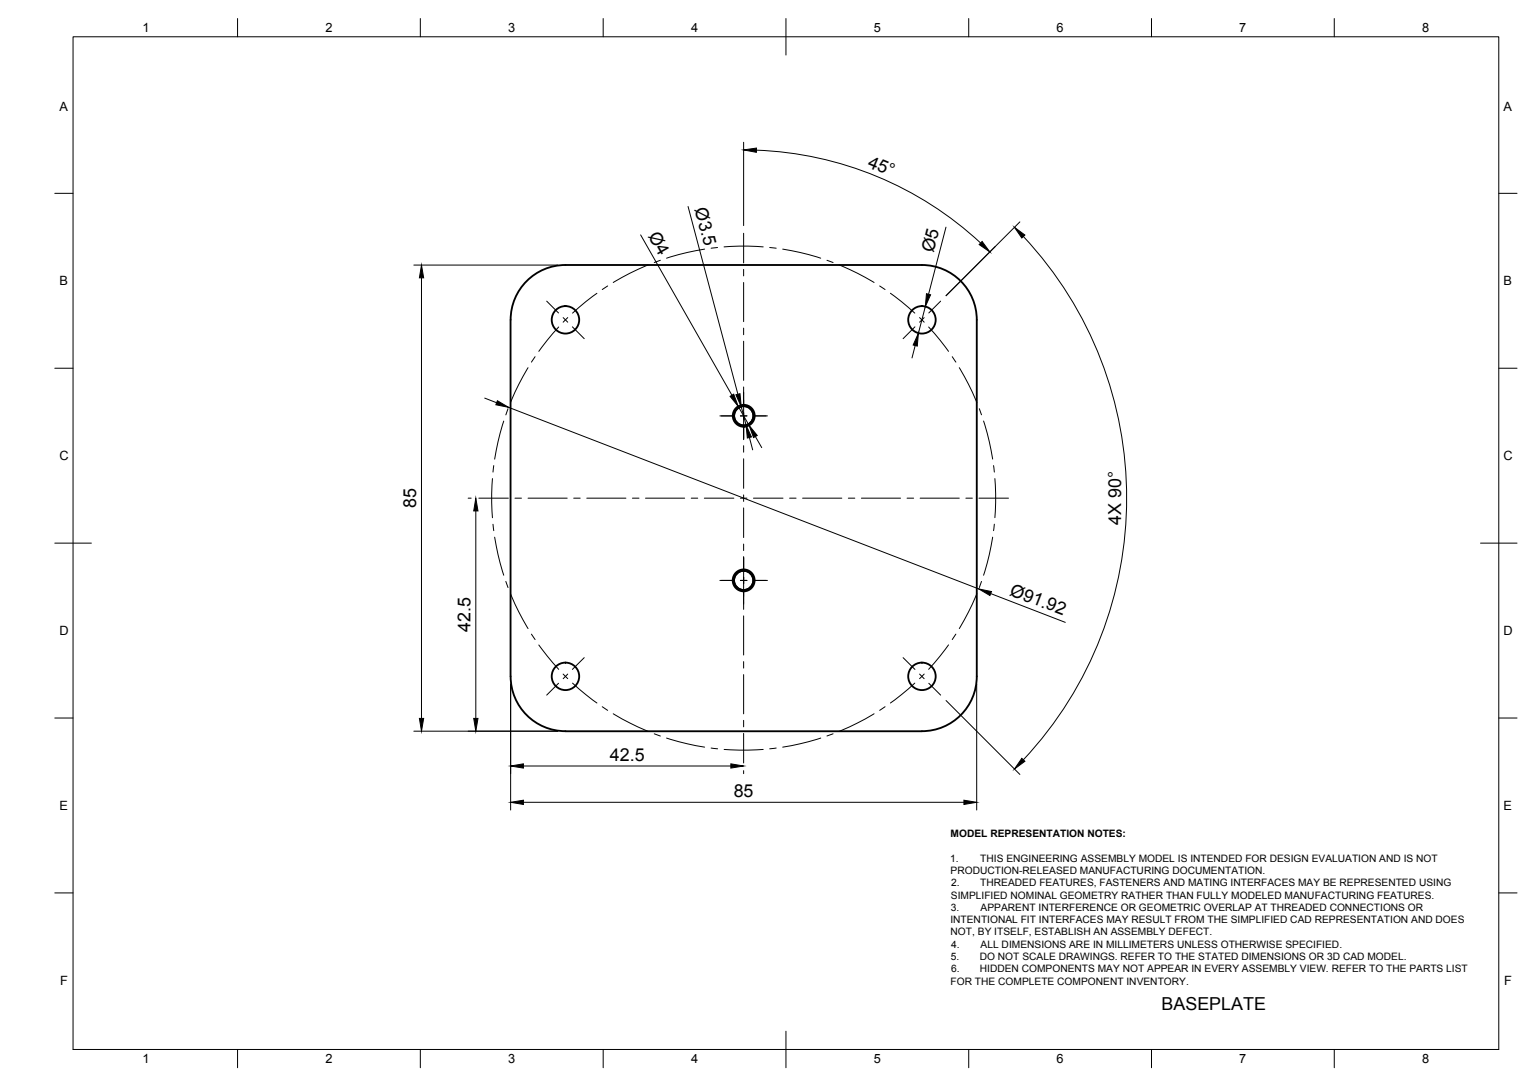
ISO-10303-21;
HEADER;
/* Generated by software containing ST-Developer
 * from STEP Tools, Inc. (www.steptools.com) 
 */

FILE_DESCRIPTION(
/* description */ (''),
/* implementation_level */ '2;1');

FILE_NAME(
/* name */ 'BASEPLATE.step',
/* time_stamp */ '2026-10-06T01:16:10-07:00',
/* author */ (''),
/* organization */ (''),
/* preprocessor_version */ 'ST-DEVELOPER v20.2',
/* originating_system */ 'Autodesk Translation Framework v15.15.0.0',
/* authorisation */ '');

FILE_SCHEMA (('AUTOMOTIVE_DESIGN { 1 0 10303 214 3 1 1 }'));
ENDSEC;

DATA;
#10=MECHANICAL_DESIGN_GEOMETRIC_PRESENTATION_REPRESENTATION('',(#297,#298,#299),#17113);
#221=OPEN_SHELL('',(#5698,#5699));
#222=OPEN_SHELL('',(#5700,#5701));
#239=SHELL_BASED_SURFACE_MODEL('Body2',(#221));
#240=SHELL_BASED_SURFACE_MODEL('Body3',(#222));
#257=CONICAL_SURFACE('',#6271,8.999999999749,0.785398163397448);
#258=CONICAL_SURFACE('',#6274,8.999999999749,0.785398163397448);
#259=CONICAL_SURFACE('',#6277,8.999999999749,0.785398163397448);
#260=CONICAL_SURFACE('',#6280,8.999999999749,0.785398163397448);
#265=SHAPE_REPRESENTATION_RELATIONSHIP('SRR','None',#17187,#281);
#281=ADVANCED_BREP_SHAPE_REPRESENTATION('',(#331),#17094);
#297=STYLED_ITEM('',(#17298),#331);
#298=STYLED_ITEM('',(#17298),#239);
#299=STYLED_ITEM('',(#17298),#240);
#331=MANIFOLD_SOLID_BREP('Body1',#6017);
#352=CYLINDRICAL_SURFACE('',#6254,2.5);
#353=CYLINDRICAL_SURFACE('',#6266,2.5);
#354=CYLINDRICAL_SURFACE('',#6267,2.5);
#355=CYLINDRICAL_SURFACE('',#6268,2.5);
#356=CYLINDRICAL_SURFACE('',#6269,1.75);
#357=CYLINDRICAL_SURFACE('',#6270,1.75);
#358=CYLINDRICAL_SURFACE('',#6284,10.);
#359=CYLINDRICAL_SURFACE('',#6286,10.);
#360=CYLINDRICAL_SURFACE('',#6288,10.);
#361=CYLINDRICAL_SURFACE('',#6290,10.);
#362=CYLINDRICAL_SURFACE('',#6291,2.);
#363=CYLINDRICAL_SURFACE('',#6296,2.);
#514=FACE_BOUND('',#1397,.T.);
#515=FACE_BOUND('',#1398,.T.);
#516=FACE_BOUND('',#1399,.T.);
#517=FACE_BOUND('',#1400,.T.);
#518=FACE_BOUND('',#1401,.T.);
#519=FACE_BOUND('',#1402,.T.);
#520=FACE_BOUND('',#1405,.T.);
#521=FACE_BOUND('',#1406,.T.);
#522=FACE_BOUND('',#1407,.T.);
#523=FACE_BOUND('',#1408,.T.);
#524=FACE_BOUND('',#1409,.T.);
#525=FACE_BOUND('',#1410,.T.);
#526=FACE_BOUND('',#1434,.T.);
#527=FACE_BOUND('',#1437,.T.);
#648=CIRCLE('',#6244,10.);
#649=CIRCLE('',#6245,10.);
#650=CIRCLE('',#6246,10.);
#651=CIRCLE('',#6247,10.);
#652=CIRCLE('',#6248,2.5);
#653=CIRCLE('',#6249,2.5);
#654=CIRCLE('',#6250,2.5);
#655=CIRCLE('',#6251,1.75);
#656=CIRCLE('',#6252,1.75);
#657=CIRCLE('',#6253,2.5);
#658=CIRCLE('',#6255,2.5);
#659=CIRCLE('',#6257,8.);
#660=CIRCLE('',#6258,8.);
#661=CIRCLE('',#6259,8.);
#662=CIRCLE('',#6260,8.);
#663=CIRCLE('',#6261,2.5);
#664=CIRCLE('',#6262,2.5);
#665=CIRCLE('',#6263,2.5);
#666=CIRCLE('',#6264,1.75);
#667=CIRCLE('',#6265,1.75);
#668=CIRCLE('',#6272,10.);
#669=CIRCLE('',#6275,10.);
#670=CIRCLE('',#6278,10.);
#671=CIRCLE('',#6281,10.);
#672=CIRCLE('',#6292,2.);
#673=CIRCLE('',#6293,2.);
#674=CIRCLE('',#6295,1.75);
#675=CIRCLE('',#6297,2.);
#676=CIRCLE('',#6298,2.);
#677=CIRCLE('',#6300,1.75);
#1026=FACE_OUTER_BOUND('',#1396,.T.);
#1027=FACE_OUTER_BOUND('',#1403,.T.);
#1028=FACE_OUTER_BOUND('',#1404,.T.);
#1029=FACE_OUTER_BOUND('',#1411,.T.);
#1030=FACE_OUTER_BOUND('',#1412,.T.);
#1031=FACE_OUTER_BOUND('',#1413,.T.);
#1032=FACE_OUTER_BOUND('',#1414,.T.);
#1033=FACE_OUTER_BOUND('',#1415,.T.);
#1034=FACE_OUTER_BOUND('',#1416,.T.);
#1035=FACE_OUTER_BOUND('',#1417,.T.);
#1036=FACE_OUTER_BOUND('',#1418,.T.);
#1037=FACE_OUTER_BOUND('',#1419,.T.);
#1038=FACE_OUTER_BOUND('',#1420,.T.);
#1039=FACE_OUTER_BOUND('',#1421,.T.);
#1040=FACE_OUTER_BOUND('',#1422,.T.);
#1041=FACE_OUTER_BOUND('',#1423,.T.);
#1042=FACE_OUTER_BOUND('',#1424,.T.);
#1043=FACE_OUTER_BOUND('',#1425,.T.);
#1044=FACE_OUTER_BOUND('',#1426,.T.);
#1045=FACE_OUTER_BOUND('',#1427,.T.);
#1046=FACE_OUTER_BOUND('',#1428,.T.);
#1047=FACE_OUTER_BOUND('',#1429,.T.);
#1048=FACE_OUTER_BOUND('',#1430,.T.);
#1049=FACE_OUTER_BOUND('',#1431,.T.);
#1050=FACE_OUTER_BOUND('',#1432,.T.);
#1051=FACE_OUTER_BOUND('',#1433,.T.);
#1052=FACE_OUTER_BOUND('',#1435,.T.);
#1053=FACE_OUTER_BOUND('',#1436,.T.);
#1396=EDGE_LOOP('',(#3996,#3997,#3998,#3999,#4000,#4001,#4002,#4003));
#1397=EDGE_LOOP('',(#4004));
#1398=EDGE_LOOP('',(#4005));
#1399=EDGE_LOOP('',(#4006));
#1400=EDGE_LOOP('',(#4007));
#1401=EDGE_LOOP('',(#4008));
#1402=EDGE_LOOP('',(#4009));
#1403=EDGE_LOOP('',(#4010,#4011,#4012,#4013));
#1404=EDGE_LOOP('',(#4014,#4015,#4016,#4017,#4018,#4019,#4020,#4021));
#1405=EDGE_LOOP('',(#4022));
#1406=EDGE_LOOP('',(#4023));
#1407=EDGE_LOOP('',(#4024));
#1408=EDGE_LOOP('',(#4025));
#1409=EDGE_LOOP('',(#4026));
#1410=EDGE_LOOP('',(#4027));
#1411=EDGE_LOOP('',(#4028,#4029,#4030,#4031));
#1412=EDGE_LOOP('',(#4032,#4033,#4034,#4035));
#1413=EDGE_LOOP('',(#4036,#4037,#4038,#4039));
#1414=EDGE_LOOP('',(#4040,#4041,#4042,#4043));
#1415=EDGE_LOOP('',(#4044,#4045,#4046,#4047));
#1416=EDGE_LOOP('',(#4048,#4049,#4050,#4051));
#1417=EDGE_LOOP('',(#4052,#4053,#4054,#4055));
#1418=EDGE_LOOP('',(#4056,#4057,#4058,#4059));
#1419=EDGE_LOOP('',(#4060,#4061,#4062,#4063));
#1420=EDGE_LOOP('',(#4064,#4065,#4066,#4067));
#1421=EDGE_LOOP('',(#4068,#4069,#4070,#4071));
#1422=EDGE_LOOP('',(#4072,#4073,#4074,#4075));
#1423=EDGE_LOOP('',(#4076,#4077,#4078,#4079));
#1424=EDGE_LOOP('',(#4080,#4081,#4082,#4083));
#1425=EDGE_LOOP('',(#4084,#4085,#4086,#4087));
#1426=EDGE_LOOP('',(#4088,#4089,#4090,#4091));
#1427=EDGE_LOOP('',(#4092,#4093,#4094,#4095));
#1428=EDGE_LOOP('',(#4096,#4097,#4098,#4099));
#1429=EDGE_LOOP('',(#4100,#4101,#4102,#4103));
#1430=EDGE_LOOP('',(#4104,#4105,#4106,#4107));
#1431=EDGE_LOOP('',(#4108,#4109,#4110,#4111));
#1432=EDGE_LOOP('',(#4112,#4113,#4114,#4115));
#1433=EDGE_LOOP('',(#4116));
#1434=EDGE_LOOP('',(#4117));
#1435=EDGE_LOOP('',(#4118,#4119,#4120,#4121));
#1436=EDGE_LOOP('',(#4122));
#1437=EDGE_LOOP('',(#4123));
#1888=LINE('',#8970,#2249);
#1889=LINE('',#8974,#2250);
#1890=LINE('',#8978,#2251);
#1891=LINE('',#8981,#2252);
#1892=LINE('',#8996,#2253);
#1893=LINE('',#9003,#2254);
#1894=LINE('',#9007,#2255);
#1895=LINE('',#9011,#2256);
#1896=LINE('',#9014,#2257);
#1897=LINE('',#9026,#2258);
#1898=LINE('',#9028,#2259);
#1899=LINE('',#9030,#2260);
#1900=LINE('',#9032,#2261);
#1901=LINE('',#9034,#2262);
#1902=LINE('',#9037,#2263);
#1903=LINE('',#9040,#2264);
#1904=LINE('',#9043,#2265);
#1905=LINE('',#9044,#2266);
#1906=LINE('',#9048,#2267);
#1907=LINE('',#9051,#2268);
#1908=LINE('',#9052,#2269);
#1909=LINE('',#9056,#2270);
#1910=LINE('',#9059,#2271);
#1911=LINE('',#9060,#2272);
#1912=LINE('',#9064,#2273);
#1913=LINE('',#9066,#2274);
#1914=LINE('',#9068,#2275);
#1915=LINE('',#9069,#2276);
#1916=LINE('',#9071,#2277);
#1917=LINE('',#9073,#2278);
#1918=LINE('',#9075,#2279);
#1919=LINE('',#9077,#2280);
#1920=LINE('',#9079,#2281);
#1921=LINE('',#9081,#2282);
#1922=LINE('',#9087,#2283);
#1923=LINE('',#9096,#2284);
#2249=VECTOR('',#7078,65.);
#2250=VECTOR('',#7081,65.);
#2251=VECTOR('',#7084,65.);
#2252=VECTOR('',#7087,65.);
#2253=VECTOR('',#7102,2.5);
#2254=VECTOR('',#7109,64.99999997841);
#2255=VECTOR('',#7112,64.99999997841);
#2256=VECTOR('',#7115,64.99999997841);
#2257=VECTOR('',#7118,64.99999997841);
#2258=VECTOR('',#7131,2.5);
#2259=VECTOR('',#7134,2.5);
#2260=VECTOR('',#7137,2.5);
#2261=VECTOR('',#7140,1.75);
#2262=VECTOR('',#7143,1.75);
#2263=VECTOR('',#7146,2.82842712475481);
#2264=VECTOR('',#7149,2.82842712476101);
#2265=VECTOR('',#7152,64.99999997975);
#2266=VECTOR('',#7153,2.82842712475481);
#2267=VECTOR('',#7158,2.82842712476081);
#2268=VECTOR('',#7161,64.99999997975);
#2269=VECTOR('',#7162,2.82842712475481);
#2270=VECTOR('',#7167,2.82842712476101);
#2271=VECTOR('',#7170,64.99999997975);
#2272=VECTOR('',#7171,2.82842712475481);
#2273=VECTOR('',#7176,2.82842712476081);
#2274=VECTOR('',#7179,64.99999997975);
#2275=VECTOR('',#7182,4.000000000157);
#2276=VECTOR('',#7183,4.00000000009);
#2277=VECTOR('',#7186,4.000000000157);
#2278=VECTOR('',#7189,4.00000000009);
#2279=VECTOR('',#7192,4.000000000157);
#2280=VECTOR('',#7195,4.00000000009);
#2281=VECTOR('',#7198,4.000000000157);
#2282=VECTOR('',#7201,4.00000000009);
#2283=VECTOR('',#7208,2.);
#2284=VECTOR('',#7219,2.);
#2608=VERTEX_POINT('',#8966);
#2609=VERTEX_POINT('',#8967);
#2610=VERTEX_POINT('',#8969);
#2611=VERTEX_POINT('',#8971);
#2612=VERTEX_POINT('',#8973);
#2613=VERTEX_POINT('',#8975);
#2614=VERTEX_POINT('',#8977);
#2615=VERTEX_POINT('',#8979);
#2616=VERTEX_POINT('',#8982);
#2617=VERTEX_POINT('',#8984);
#2618=VERTEX_POINT('',#8986);
#2619=VERTEX_POINT('',#8988);
#2620=VERTEX_POINT('',#8990);
#2621=VERTEX_POINT('',#8992);
#2622=VERTEX_POINT('',#8995);
#2623=VERTEX_POINT('',#8999);
#2624=VERTEX_POINT('',#9000);
#2625=VERTEX_POINT('',#9002);
#2626=VERTEX_POINT('',#9004);
#2627=VERTEX_POINT('',#9006);
#2628=VERTEX_POINT('',#9008);
#2629=VERTEX_POINT('',#9010);
#2630=VERTEX_POINT('',#9012);
#2631=VERTEX_POINT('',#9015);
#2632=VERTEX_POINT('',#9017);
#2633=VERTEX_POINT('',#9019);
#2634=VERTEX_POINT('',#9021);
#2635=VERTEX_POINT('',#9023);
#2636=VERTEX_POINT('',#9036);
#2637=VERTEX_POINT('',#9038);
#2638=VERTEX_POINT('',#9042);
#2639=VERTEX_POINT('',#9046);
#2640=VERTEX_POINT('',#9050);
#2641=VERTEX_POINT('',#9054);
#2642=VERTEX_POINT('',#9058);
#2643=VERTEX_POINT('',#9062);
#2644=VERTEX_POINT('',#9084);
#2645=VERTEX_POINT('',#9086);
#2646=VERTEX_POINT('',#9090);
#2647=VERTEX_POINT('',#9093);
#2648=VERTEX_POINT('',#9095);
#2649=VERTEX_POINT('',#9099);
#3144=EDGE_CURVE('',#2608,#2609,#648,.T.);
#3145=EDGE_CURVE('',#2610,#2608,#1888,.T.);
#3146=EDGE_CURVE('',#2611,#2610,#649,.T.);
#3147=EDGE_CURVE('',#2612,#2611,#1889,.T.);
#3148=EDGE_CURVE('',#2613,#2612,#650,.T.);
#3149=EDGE_CURVE('',#2614,#2613,#1890,.T.);
#3150=EDGE_CURVE('',#2615,#2614,#651,.T.);
#3151=EDGE_CURVE('',#2609,#2615,#1891,.T.);
#3152=EDGE_CURVE('',#2616,#2616,#652,.T.);
#3153=EDGE_CURVE('',#2617,#2617,#653,.T.);
#3154=EDGE_CURVE('',#2618,#2618,#654,.T.);
#3155=EDGE_CURVE('',#2619,#2619,#655,.T.);
#3156=EDGE_CURVE('',#2620,#2620,#656,.T.);
#3157=EDGE_CURVE('',#2621,#2621,#657,.T.);
#3158=EDGE_CURVE('',#2621,#2622,#1892,.T.);
#3159=EDGE_CURVE('',#2622,#2622,#658,.T.);
#3160=EDGE_CURVE('',#2623,#2624,#659,.T.);
#3161=EDGE_CURVE('',#2624,#2625,#1893,.T.);
#3162=EDGE_CURVE('',#2625,#2626,#660,.T.);
#3163=EDGE_CURVE('',#2626,#2627,#1894,.T.);
#3164=EDGE_CURVE('',#2627,#2628,#661,.T.);
#3165=EDGE_CURVE('',#2628,#2629,#1895,.T.);
#3166=EDGE_CURVE('',#2629,#2630,#662,.T.);
#3167=EDGE_CURVE('',#2630,#2623,#1896,.T.);
#3168=EDGE_CURVE('',#2631,#2631,#663,.T.);
#3169=EDGE_CURVE('',#2632,#2632,#664,.T.);
#3170=EDGE_CURVE('',#2633,#2633,#665,.T.);
#3171=EDGE_CURVE('',#2634,#2634,#666,.T.);
#3172=EDGE_CURVE('',#2635,#2635,#667,.T.);
#3173=EDGE_CURVE('',#2616,#2631,#1897,.T.);
#3174=EDGE_CURVE('',#2617,#2632,#1898,.T.);
#3175=EDGE_CURVE('',#2618,#2633,#1899,.T.);
#3176=EDGE_CURVE('',#2619,#2634,#1900,.T.);
#3177=EDGE_CURVE('',#2620,#2635,#1901,.T.);
#3178=EDGE_CURVE('',#2623,#2636,#1902,.T.);
#3179=EDGE_CURVE('',#2636,#2637,#668,.T.);
#3180=EDGE_CURVE('',#2624,#2637,#1903,.T.);
#3181=EDGE_CURVE('',#2637,#2638,#1904,.T.);
#3182=EDGE_CURVE('',#2625,#2638,#1905,.T.);
#3183=EDGE_CURVE('',#2638,#2639,#669,.T.);
#3184=EDGE_CURVE('',#2626,#2639,#1906,.T.);
#3185=EDGE_CURVE('',#2639,#2640,#1907,.T.);
#3186=EDGE_CURVE('',#2627,#2640,#1908,.T.);
#3187=EDGE_CURVE('',#2640,#2641,#670,.T.);
#3188=EDGE_CURVE('',#2628,#2641,#1909,.T.);
#3189=EDGE_CURVE('',#2641,#2642,#1910,.T.);
#3190=EDGE_CURVE('',#2629,#2642,#1911,.T.);
#3191=EDGE_CURVE('',#2642,#2643,#671,.T.);
#3192=EDGE_CURVE('',#2630,#2643,#1912,.T.);
#3193=EDGE_CURVE('',#2643,#2636,#1913,.T.);
#3194=EDGE_CURVE('',#2612,#2643,#1914,.T.);
#3195=EDGE_CURVE('',#2611,#2636,#1915,.T.);
#3196=EDGE_CURVE('',#2610,#2637,#1916,.T.);
#3197=EDGE_CURVE('',#2608,#2638,#1917,.T.);
#3198=EDGE_CURVE('',#2609,#2639,#1918,.T.);
#3199=EDGE_CURVE('',#2615,#2640,#1919,.T.);
#3200=EDGE_CURVE('',#2614,#2641,#1920,.T.);
#3201=EDGE_CURVE('',#2613,#2642,#1921,.T.);
#3202=EDGE_CURVE('',#2644,#2644,#672,.T.);
#3203=EDGE_CURVE('',#2644,#2645,#1922,.T.);
#3204=EDGE_CURVE('',#2645,#2645,#673,.T.);
#3205=EDGE_CURVE('',#2646,#2646,#674,.T.);
#3206=EDGE_CURVE('',#2647,#2647,#675,.T.);
#3207=EDGE_CURVE('',#2647,#2648,#1923,.T.);
#3208=EDGE_CURVE('',#2648,#2648,#676,.T.);
#3209=EDGE_CURVE('',#2649,#2649,#677,.T.);
#3996=ORIENTED_EDGE('',*,*,#3144,.F.);
#3997=ORIENTED_EDGE('',*,*,#3145,.F.);
#3998=ORIENTED_EDGE('',*,*,#3146,.F.);
#3999=ORIENTED_EDGE('',*,*,#3147,.F.);
#4000=ORIENTED_EDGE('',*,*,#3148,.F.);
#4001=ORIENTED_EDGE('',*,*,#3149,.F.);
#4002=ORIENTED_EDGE('',*,*,#3150,.F.);
#4003=ORIENTED_EDGE('',*,*,#3151,.F.);
#4004=ORIENTED_EDGE('',*,*,#3152,.F.);
#4005=ORIENTED_EDGE('',*,*,#3153,.F.);
#4006=ORIENTED_EDGE('',*,*,#3154,.F.);
#4007=ORIENTED_EDGE('',*,*,#3155,.F.);
#4008=ORIENTED_EDGE('',*,*,#3156,.F.);
#4009=ORIENTED_EDGE('',*,*,#3157,.F.);
#4010=ORIENTED_EDGE('',*,*,#3157,.T.);
#4011=ORIENTED_EDGE('',*,*,#3158,.T.);
#4012=ORIENTED_EDGE('',*,*,#3159,.F.);
#4013=ORIENTED_EDGE('',*,*,#3158,.F.);
#4014=ORIENTED_EDGE('',*,*,#3160,.T.);
#4015=ORIENTED_EDGE('',*,*,#3161,.T.);
#4016=ORIENTED_EDGE('',*,*,#3162,.T.);
#4017=ORIENTED_EDGE('',*,*,#3163,.T.);
#4018=ORIENTED_EDGE('',*,*,#3164,.T.);
#4019=ORIENTED_EDGE('',*,*,#3165,.T.);
#4020=ORIENTED_EDGE('',*,*,#3166,.T.);
#4021=ORIENTED_EDGE('',*,*,#3167,.T.);
#4022=ORIENTED_EDGE('',*,*,#3168,.T.);
#4023=ORIENTED_EDGE('',*,*,#3169,.T.);
#4024=ORIENTED_EDGE('',*,*,#3170,.T.);
#4025=ORIENTED_EDGE('',*,*,#3171,.T.);
#4026=ORIENTED_EDGE('',*,*,#3172,.T.);
#4027=ORIENTED_EDGE('',*,*,#3159,.T.);
#4028=ORIENTED_EDGE('',*,*,#3152,.T.);
#4029=ORIENTED_EDGE('',*,*,#3173,.T.);
#4030=ORIENTED_EDGE('',*,*,#3168,.F.);
#4031=ORIENTED_EDGE('',*,*,#3173,.F.);
#4032=ORIENTED_EDGE('',*,*,#3153,.T.);
#4033=ORIENTED_EDGE('',*,*,#3174,.T.);
#4034=ORIENTED_EDGE('',*,*,#3169,.F.);
#4035=ORIENTED_EDGE('',*,*,#3174,.F.);
#4036=ORIENTED_EDGE('',*,*,#3154,.T.);
#4037=ORIENTED_EDGE('',*,*,#3175,.T.);
#4038=ORIENTED_EDGE('',*,*,#3170,.F.);
#4039=ORIENTED_EDGE('',*,*,#3175,.F.);
#4040=ORIENTED_EDGE('',*,*,#3155,.T.);
#4041=ORIENTED_EDGE('',*,*,#3176,.T.);
#4042=ORIENTED_EDGE('',*,*,#3171,.F.);
#4043=ORIENTED_EDGE('',*,*,#3176,.F.);
#4044=ORIENTED_EDGE('',*,*,#3156,.T.);
#4045=ORIENTED_EDGE('',*,*,#3177,.T.);
#4046=ORIENTED_EDGE('',*,*,#3172,.F.);
#4047=ORIENTED_EDGE('',*,*,#3177,.F.);
#4048=ORIENTED_EDGE('',*,*,#3160,.F.);
#4049=ORIENTED_EDGE('',*,*,#3178,.T.);
#4050=ORIENTED_EDGE('',*,*,#3179,.T.);
#4051=ORIENTED_EDGE('',*,*,#3180,.F.);
#4052=ORIENTED_EDGE('',*,*,#3161,.F.);
#4053=ORIENTED_EDGE('',*,*,#3180,.T.);
#4054=ORIENTED_EDGE('',*,*,#3181,.T.);
#4055=ORIENTED_EDGE('',*,*,#3182,.F.);
#4056=ORIENTED_EDGE('',*,*,#3162,.F.);
#4057=ORIENTED_EDGE('',*,*,#3182,.T.);
#4058=ORIENTED_EDGE('',*,*,#3183,.T.);
#4059=ORIENTED_EDGE('',*,*,#3184,.F.);
#4060=ORIENTED_EDGE('',*,*,#3163,.F.);
#4061=ORIENTED_EDGE('',*,*,#3184,.T.);
#4062=ORIENTED_EDGE('',*,*,#3185,.T.);
#4063=ORIENTED_EDGE('',*,*,#3186,.F.);
#4064=ORIENTED_EDGE('',*,*,#3164,.F.);
#4065=ORIENTED_EDGE('',*,*,#3186,.T.);
#4066=ORIENTED_EDGE('',*,*,#3187,.T.);
#4067=ORIENTED_EDGE('',*,*,#3188,.F.);
#4068=ORIENTED_EDGE('',*,*,#3165,.F.);
#4069=ORIENTED_EDGE('',*,*,#3188,.T.);
#4070=ORIENTED_EDGE('',*,*,#3189,.T.);
#4071=ORIENTED_EDGE('',*,*,#3190,.F.);
#4072=ORIENTED_EDGE('',*,*,#3166,.F.);
#4073=ORIENTED_EDGE('',*,*,#3190,.T.);
#4074=ORIENTED_EDGE('',*,*,#3191,.T.);
#4075=ORIENTED_EDGE('',*,*,#3192,.F.);
#4076=ORIENTED_EDGE('',*,*,#3167,.F.);
#4077=ORIENTED_EDGE('',*,*,#3192,.T.);
#4078=ORIENTED_EDGE('',*,*,#3193,.T.);
#4079=ORIENTED_EDGE('',*,*,#3178,.F.);
#4080=ORIENTED_EDGE('',*,*,#3193,.F.);
#4081=ORIENTED_EDGE('',*,*,#3194,.F.);
#4082=ORIENTED_EDGE('',*,*,#3147,.T.);
#4083=ORIENTED_EDGE('',*,*,#3195,.T.);
#4084=ORIENTED_EDGE('',*,*,#3179,.F.);
#4085=ORIENTED_EDGE('',*,*,#3195,.F.);
#4086=ORIENTED_EDGE('',*,*,#3146,.T.);
#4087=ORIENTED_EDGE('',*,*,#3196,.T.);
#4088=ORIENTED_EDGE('',*,*,#3181,.F.);
#4089=ORIENTED_EDGE('',*,*,#3196,.F.);
#4090=ORIENTED_EDGE('',*,*,#3145,.T.);
#4091=ORIENTED_EDGE('',*,*,#3197,.T.);
#4092=ORIENTED_EDGE('',*,*,#3183,.F.);
#4093=ORIENTED_EDGE('',*,*,#3197,.F.);
#4094=ORIENTED_EDGE('',*,*,#3144,.T.);
#4095=ORIENTED_EDGE('',*,*,#3198,.T.);
#4096=ORIENTED_EDGE('',*,*,#3185,.F.);
#4097=ORIENTED_EDGE('',*,*,#3198,.F.);
#4098=ORIENTED_EDGE('',*,*,#3151,.T.);
#4099=ORIENTED_EDGE('',*,*,#3199,.T.);
#4100=ORIENTED_EDGE('',*,*,#3187,.F.);
#4101=ORIENTED_EDGE('',*,*,#3199,.F.);
#4102=ORIENTED_EDGE('',*,*,#3150,.T.);
#4103=ORIENTED_EDGE('',*,*,#3200,.T.);
#4104=ORIENTED_EDGE('',*,*,#3189,.F.);
#4105=ORIENTED_EDGE('',*,*,#3200,.F.);
#4106=ORIENTED_EDGE('',*,*,#3149,.T.);
#4107=ORIENTED_EDGE('',*,*,#3201,.T.);
#4108=ORIENTED_EDGE('',*,*,#3191,.F.);
#4109=ORIENTED_EDGE('',*,*,#3201,.F.);
#4110=ORIENTED_EDGE('',*,*,#3148,.T.);
#4111=ORIENTED_EDGE('',*,*,#3194,.T.);
#4112=ORIENTED_EDGE('',*,*,#3202,.F.);
#4113=ORIENTED_EDGE('',*,*,#3203,.T.);
#4114=ORIENTED_EDGE('',*,*,#3204,.T.);
#4115=ORIENTED_EDGE('',*,*,#3203,.F.);
#4116=ORIENTED_EDGE('',*,*,#3204,.F.);
#4117=ORIENTED_EDGE('',*,*,#3205,.F.);
#4118=ORIENTED_EDGE('',*,*,#3206,.F.);
#4119=ORIENTED_EDGE('',*,*,#3207,.T.);
#4120=ORIENTED_EDGE('',*,*,#3208,.T.);
#4121=ORIENTED_EDGE('',*,*,#3207,.F.);
#4122=ORIENTED_EDGE('',*,*,#3208,.F.);
#4123=ORIENTED_EDGE('',*,*,#3209,.F.);
#5516=PLANE('',#6243);
#5517=PLANE('',#6256);
#5518=PLANE('',#6273);
#5519=PLANE('',#6276);
#5520=PLANE('',#6279);
#5521=PLANE('',#6282);
#5522=PLANE('',#6283);
#5523=PLANE('',#6285);
#5524=PLANE('',#6287);
#5525=PLANE('',#6289);
#5526=PLANE('',#6294);
#5527=PLANE('',#6299);
#5674=ADVANCED_FACE('',(#1026,#514,#515,#516,#517,#518,#519),#5516,.F.);
#5675=ADVANCED_FACE('',(#1027),#352,.F.);
#5676=ADVANCED_FACE('',(#1028,#520,#521,#522,#523,#524,#525),#5517,.T.);
#5677=ADVANCED_FACE('',(#1029),#353,.F.);
#5678=ADVANCED_FACE('',(#1030),#354,.F.);
#5679=ADVANCED_FACE('',(#1031),#355,.F.);
#5680=ADVANCED_FACE('',(#1032),#356,.F.);
#5681=ADVANCED_FACE('',(#1033),#357,.F.);
#5682=ADVANCED_FACE('',(#1034),#257,.T.);
#5683=ADVANCED_FACE('',(#1035),#5518,.T.);
#5684=ADVANCED_FACE('',(#1036),#258,.T.);
#5685=ADVANCED_FACE('',(#1037),#5519,.T.);
#5686=ADVANCED_FACE('',(#1038),#259,.T.);
#5687=ADVANCED_FACE('',(#1039),#5520,.T.);
#5688=ADVANCED_FACE('',(#1040),#260,.T.);
#5689=ADVANCED_FACE('',(#1041),#5521,.T.);
#5690=ADVANCED_FACE('',(#1042),#5522,.T.);
#5691=ADVANCED_FACE('',(#1043),#358,.T.);
#5692=ADVANCED_FACE('',(#1044),#5523,.T.);
#5693=ADVANCED_FACE('',(#1045),#359,.T.);
#5694=ADVANCED_FACE('',(#1046),#5524,.T.);
#5695=ADVANCED_FACE('',(#1047),#360,.T.);
#5696=ADVANCED_FACE('',(#1048),#5525,.T.);
#5697=ADVANCED_FACE('',(#1049),#361,.T.);
#5698=ADVANCED_FACE('',(#1050),#362,.T.);
#5699=ADVANCED_FACE('',(#1051,#526),#5526,.F.);
#5700=ADVANCED_FACE('',(#1052),#363,.T.);
#5701=ADVANCED_FACE('',(#1053,#527),#5527,.F.);
#6017=CLOSED_SHELL('',(#5674,#5675,#5676,#5677,#5678,#5679,#5680,#5681,
#5682,#5683,#5684,#5685,#5686,#5687,#5688,#5689,#5690,#5691,#5692,#5693,
#5694,#5695,#5696,#5697));
#6242=AXIS2_PLACEMENT_3D('',#8964,#7072,#7073);
#6243=AXIS2_PLACEMENT_3D('',#8965,#7074,#7075);
#6244=AXIS2_PLACEMENT_3D('',#8968,#7076,#7077);
#6245=AXIS2_PLACEMENT_3D('',#8972,#7079,#7080);
#6246=AXIS2_PLACEMENT_3D('',#8976,#7082,#7083);
#6247=AXIS2_PLACEMENT_3D('',#8980,#7085,#7086);
#6248=AXIS2_PLACEMENT_3D('',#8983,#7088,#7089);
#6249=AXIS2_PLACEMENT_3D('',#8985,#7090,#7091);
#6250=AXIS2_PLACEMENT_3D('',#8987,#7092,#7093);
#6251=AXIS2_PLACEMENT_3D('',#8989,#7094,#7095);
#6252=AXIS2_PLACEMENT_3D('',#8991,#7096,#7097);
#6253=AXIS2_PLACEMENT_3D('',#8993,#7098,#7099);
#6254=AXIS2_PLACEMENT_3D('',#8994,#7100,#7101);
#6255=AXIS2_PLACEMENT_3D('',#8997,#7103,#7104);
#6256=AXIS2_PLACEMENT_3D('',#8998,#7105,#7106);
#6257=AXIS2_PLACEMENT_3D('',#9001,#7107,#7108);
#6258=AXIS2_PLACEMENT_3D('',#9005,#7110,#7111);
#6259=AXIS2_PLACEMENT_3D('',#9009,#7113,#7114);
#6260=AXIS2_PLACEMENT_3D('',#9013,#7116,#7117);
#6261=AXIS2_PLACEMENT_3D('',#9016,#7119,#7120);
#6262=AXIS2_PLACEMENT_3D('',#9018,#7121,#7122);
#6263=AXIS2_PLACEMENT_3D('',#9020,#7123,#7124);
#6264=AXIS2_PLACEMENT_3D('',#9022,#7125,#7126);
#6265=AXIS2_PLACEMENT_3D('',#9024,#7127,#7128);
#6266=AXIS2_PLACEMENT_3D('',#9025,#7129,#7130);
#6267=AXIS2_PLACEMENT_3D('',#9027,#7132,#7133);
#6268=AXIS2_PLACEMENT_3D('',#9029,#7135,#7136);
#6269=AXIS2_PLACEMENT_3D('',#9031,#7138,#7139);
#6270=AXIS2_PLACEMENT_3D('',#9033,#7141,#7142);
#6271=AXIS2_PLACEMENT_3D('',#9035,#7144,#7145);
#6272=AXIS2_PLACEMENT_3D('',#9039,#7147,#7148);
#6273=AXIS2_PLACEMENT_3D('',#9041,#7150,#7151);
#6274=AXIS2_PLACEMENT_3D('',#9045,#7154,#7155);
#6275=AXIS2_PLACEMENT_3D('',#9047,#7156,#7157);
#6276=AXIS2_PLACEMENT_3D('',#9049,#7159,#7160);
#6277=AXIS2_PLACEMENT_3D('',#9053,#7163,#7164);
#6278=AXIS2_PLACEMENT_3D('',#9055,#7165,#7166);
#6279=AXIS2_PLACEMENT_3D('',#9057,#7168,#7169);
#6280=AXIS2_PLACEMENT_3D('',#9061,#7172,#7173);
#6281=AXIS2_PLACEMENT_3D('',#9063,#7174,#7175);
#6282=AXIS2_PLACEMENT_3D('',#9065,#7177,#7178);
#6283=AXIS2_PLACEMENT_3D('',#9067,#7180,#7181);
#6284=AXIS2_PLACEMENT_3D('',#9070,#7184,#7185);
#6285=AXIS2_PLACEMENT_3D('',#9072,#7187,#7188);
#6286=AXIS2_PLACEMENT_3D('',#9074,#7190,#7191);
#6287=AXIS2_PLACEMENT_3D('',#9076,#7193,#7194);
#6288=AXIS2_PLACEMENT_3D('',#9078,#7196,#7197);
#6289=AXIS2_PLACEMENT_3D('',#9080,#7199,#7200);
#6290=AXIS2_PLACEMENT_3D('',#9082,#7202,#7203);
#6291=AXIS2_PLACEMENT_3D('',#9083,#7204,#7205);
#6292=AXIS2_PLACEMENT_3D('',#9085,#7206,#7207);
#6293=AXIS2_PLACEMENT_3D('',#9088,#7209,#7210);
#6294=AXIS2_PLACEMENT_3D('',#9089,#7211,#7212);
#6295=AXIS2_PLACEMENT_3D('',#9091,#7213,#7214);
#6296=AXIS2_PLACEMENT_3D('',#9092,#7215,#7216);
#6297=AXIS2_PLACEMENT_3D('',#9094,#7217,#7218);
#6298=AXIS2_PLACEMENT_3D('',#9097,#7220,#7221);
#6299=AXIS2_PLACEMENT_3D('',#9098,#7222,#7223);
#6300=AXIS2_PLACEMENT_3D('',#9100,#7224,#7225);
#7072=DIRECTION('axis',(0.,0.,1.));
#7073=DIRECTION('refdir',(1.,0.,0.));
#7074=DIRECTION('center_axis',(0.,1.,0.));
#7075=DIRECTION('ref_axis',(1.,0.,0.));
#7076=DIRECTION('center_axis',(0.,1.,0.));
#7077=DIRECTION('ref_axis',(0.,0.,-1.));
#7078=DIRECTION('',(-1.,0.,0.));
#7079=DIRECTION('center_axis',(0.,1.,0.));
#7080=DIRECTION('ref_axis',(1.,0.,0.));
#7081=DIRECTION('',(0.,0.,-1.));
#7082=DIRECTION('center_axis',(0.,1.,0.));
#7083=DIRECTION('ref_axis',(0.,0.,1.));
#7084=DIRECTION('',(1.,0.,0.));
#7085=DIRECTION('center_axis',(0.,1.,0.));
#7086=DIRECTION('ref_axis',(-1.,0.,0.));
#7087=DIRECTION('',(0.,0.,1.));
#7088=DIRECTION('center_axis',(0.,-1.,0.));
#7089=DIRECTION('ref_axis',(1.,0.,0.));
#7090=DIRECTION('center_axis',(0.,-1.,0.));
#7091=DIRECTION('ref_axis',(1.,0.,0.));
#7092=DIRECTION('center_axis',(0.,-1.,0.));
#7093=DIRECTION('ref_axis',(1.,0.,0.));
#7094=DIRECTION('center_axis',(0.,-1.,0.));
#7095=DIRECTION('ref_axis',(1.,0.,0.));
#7096=DIRECTION('center_axis',(0.,-1.,0.));
#7097=DIRECTION('ref_axis',(1.,0.,0.));
#7098=DIRECTION('center_axis',(0.,-1.,0.));
#7099=DIRECTION('ref_axis',(1.,0.,0.));
#7100=DIRECTION('center_axis',(0.,1.,0.));
#7101=DIRECTION('ref_axis',(1.,0.,0.));
#7102=DIRECTION('',(0.,1.,0.));
#7103=DIRECTION('center_axis',(0.,-1.,0.));
#7104=DIRECTION('ref_axis',(1.,0.,0.));
#7105=DIRECTION('center_axis',(0.,1.,0.));
#7106=DIRECTION('ref_axis',(1.,0.,0.));
#7107=DIRECTION('center_axis',(0.,1.,0.));
#7108=DIRECTION('ref_axis',(1.,0.,0.));
#7109=DIRECTION('',(-1.,-1.086597479022E-12,-1.086802443273E-12));
#7110=DIRECTION('center_axis',(0.,1.,0.));
#7111=DIRECTION('ref_axis',(0.,0.,-1.));
#7112=DIRECTION('',(-1.086583814739E-12,-1.086583814739E-12,1.));
#7113=DIRECTION('center_axis',(0.,1.,0.));
#7114=DIRECTION('ref_axis',(-1.,0.,0.));
#7115=DIRECTION('',(1.,-1.086583814739E-12,1.086802443273E-12));
#7116=DIRECTION('center_axis',(0.,1.,0.));
#7117=DIRECTION('ref_axis',(0.,0.,1.));
#7118=DIRECTION('',(1.086583814739E-12,-1.086597479022E-12,-1.));
#7119=DIRECTION('center_axis',(0.,-1.,0.));
#7120=DIRECTION('ref_axis',(1.,0.,0.));
#7121=DIRECTION('center_axis',(0.,-1.,0.));
#7122=DIRECTION('ref_axis',(1.,0.,0.));
#7123=DIRECTION('center_axis',(0.,-1.,0.));
#7124=DIRECTION('ref_axis',(1.,0.,0.));
#7125=DIRECTION('center_axis',(0.,-1.,0.));
#7126=DIRECTION('ref_axis',(1.,0.,0.));
#7127=DIRECTION('center_axis',(0.,-1.,0.));
#7128=DIRECTION('ref_axis',(1.,0.,0.));
#7129=DIRECTION('center_axis',(0.,1.,0.));
#7130=DIRECTION('ref_axis',(1.,0.,0.));
#7131=DIRECTION('',(0.,1.,0.));
#7132=DIRECTION('center_axis',(0.,1.,0.));
#7133=DIRECTION('ref_axis',(1.,0.,0.));
#7134=DIRECTION('',(0.,1.,0.));
#7135=DIRECTION('center_axis',(0.,1.,0.));
#7136=DIRECTION('ref_axis',(1.,0.,0.));
#7137=DIRECTION('',(0.,1.,0.));
#7138=DIRECTION('center_axis',(0.,1.,0.));
#7139=DIRECTION('ref_axis',(1.,0.,0.));
#7140=DIRECTION('',(0.,1.,0.));
#7141=DIRECTION('center_axis',(0.,1.,0.));
#7142=DIRECTION('ref_axis',(1.,0.,0.));
#7143=DIRECTION('',(0.,1.,0.));
#7144=DIRECTION('center_axis',(0.,-1.,0.));
#7145=DIRECTION('ref_axis',(0.,0.,-1.));
#7146=DIRECTION('',(0.707106781186548,-0.707106781186548,-2.27691040135715E-10));
#7147=DIRECTION('center_axis',(0.,1.,0.));
#7148=DIRECTION('ref_axis',(1.,0.,0.));
#7149=DIRECTION('',(2.49493972053399E-10,-0.707106781186498,-0.707106781186598));
#7150=DIRECTION('center_axis',(0.,0.707106781186548,-0.707106781186548));
#7151=DIRECTION('ref_axis',(0.,-0.707106781186548,-0.707106781186548));
#7152=DIRECTION('',(-1.,-1.018672326296E-12,-1.01880896913E-12));
#7153=DIRECTION('',(-2.27688527987815E-10,-0.707106781186548,-0.707106781186548));
#7154=DIRECTION('center_axis',(0.,-1.,0.));
#7155=DIRECTION('ref_axis',(0.,0.,-1.));
#7156=DIRECTION('center_axis',(0.,1.,0.));
#7157=DIRECTION('ref_axis',(0.,0.,-1.));
#7158=DIRECTION('',(-0.707106781186548,-0.707106781186548,-2.49493972053417E-10));
#7159=DIRECTION('center_axis',(-0.707106781186548,0.707106781186548,0.));
#7160=DIRECTION('ref_axis',(-0.707106781186548,-0.707106781186548,0.));
#7161=DIRECTION('',(-1.018590340596E-12,-1.018658662013E-12,1.));
#7162=DIRECTION('',(-0.707106781186548,-0.707106781186548,2.27691040135715E-10));
#7163=DIRECTION('center_axis',(0.,-1.,0.));
#7164=DIRECTION('ref_axis',(-0.707106781142795,0.,0.7071067812303));
#7165=DIRECTION('center_axis',(0.,1.,0.));
#7166=DIRECTION('ref_axis',(-1.,0.,0.));
#7167=DIRECTION('',(-2.49493972053399E-10,-0.707106781186498,0.707106781186598));
#7168=DIRECTION('center_axis',(0.,0.707106781186548,0.707106781186548));
#7169=DIRECTION('ref_axis',(0.,-0.707106781186548,0.707106781186548));
#7170=DIRECTION('',(1.,-1.018672326296E-12,1.01880896913E-12));
#7171=DIRECTION('',(2.27688527987815E-10,-0.707106781186548,0.707106781186548));
#7172=DIRECTION('center_axis',(0.,-1.,0.));
#7173=DIRECTION('ref_axis',(0.7071067812303,0.,0.707106781142795));
#7174=DIRECTION('center_axis',(0.,1.,0.));
#7175=DIRECTION('ref_axis',(0.,0.,1.));
#7176=DIRECTION('',(0.707106781186548,-0.707106781186548,2.49496484201317E-10));
#7177=DIRECTION('center_axis',(0.707106781186548,0.707106781186548,0.));
#7178=DIRECTION('ref_axis',(0.707106781186548,-0.707106781186548,0.));
#7179=DIRECTION('',(1.018590340596E-12,-1.018672326296E-12,-1.));
#7180=DIRECTION('center_axis',(1.,0.,0.));
#7181=DIRECTION('ref_axis',(0.,0.,-1.));
#7182=DIRECTION('',(-3.916511559356E-11,1.,-2.646281416115E-9));
#7183=DIRECTION('',(-2.261124620821E-11,1.,2.415008637458E-9));
#7184=DIRECTION('center_axis',(0.,1.,0.));
#7185=DIRECTION('ref_axis',(1.,0.,0.));
#7186=DIRECTION('',(-2.646279639758E-9,1.,3.91668919504E-11));
#7187=DIRECTION('center_axis',(0.,0.,-1.));
#7188=DIRECTION('ref_axis',(-1.,0.,0.));
#7189=DIRECTION('',(2.415006861102E-9,1.,2.261124620821E-11));
#7190=DIRECTION('center_axis',(0.,1.,0.));
#7191=DIRECTION('ref_axis',(-0.707106781219254,0.,-0.707106781153841));
#7192=DIRECTION('',(3.916511559356E-11,1.,2.646279639758E-9));
#7193=DIRECTION('center_axis',(-1.,0.,0.));
#7194=DIRECTION('ref_axis',(0.,0.,1.));
#7195=DIRECTION('',(2.261124620821E-11,1.,-2.415008637458E-9));
#7196=DIRECTION('center_axis',(0.,1.,0.));
#7197=DIRECTION('ref_axis',(-0.707106781153841,0.,0.707106781219254));
#7198=DIRECTION('',(2.646279639758E-9,1.,-3.91668919504E-11));
#7199=DIRECTION('center_axis',(0.,0.,1.));
#7200=DIRECTION('ref_axis',(1.,0.,0.));
#7201=DIRECTION('',(-2.415006861102E-9,1.,-2.261124620821E-11));
#7202=DIRECTION('center_axis',(0.,1.,0.));
#7203=DIRECTION('ref_axis',(1.,0.,0.));
#7204=DIRECTION('center_axis',(0.,1.,0.));
#7205=DIRECTION('ref_axis',(-1.,0.,0.));
#7206=DIRECTION('center_axis',(0.,1.,0.));
#7207=DIRECTION('ref_axis',(1.,0.,0.));
#7208=DIRECTION('',(0.,-1.,0.));
#7209=DIRECTION('center_axis',(0.,1.,0.));
#7210=DIRECTION('ref_axis',(1.,0.,0.));
#7211=DIRECTION('center_axis',(0.,1.,0.));
#7212=DIRECTION('ref_axis',(-1.,0.,0.));
#7213=DIRECTION('center_axis',(0.,-1.,0.));
#7214=DIRECTION('ref_axis',(1.,0.,0.));
#7215=DIRECTION('center_axis',(0.,1.,0.));
#7216=DIRECTION('ref_axis',(-1.,0.,0.));
#7217=DIRECTION('center_axis',(0.,1.,0.));
#7218=DIRECTION('ref_axis',(1.,0.,0.));
#7219=DIRECTION('',(0.,-1.,0.));
#7220=DIRECTION('center_axis',(0.,1.,0.));
#7221=DIRECTION('ref_axis',(1.,0.,0.));
#7222=DIRECTION('center_axis',(0.,1.,0.));
#7223=DIRECTION('ref_axis',(-1.,0.,0.));
#7224=DIRECTION('center_axis',(0.,-1.,0.));
#7225=DIRECTION('ref_axis',(1.,0.,0.));
#8964=CARTESIAN_POINT('',(0.,0.,0.));
#8965=CARTESIAN_POINT('Origin',(0.,0.,0.));
#8966=CARTESIAN_POINT('',(-32.5,0.,-42.5));
#8967=CARTESIAN_POINT('',(-42.5,0.,-32.5));
#8968=CARTESIAN_POINT('Origin',(-32.5,0.,-32.5));
#8969=CARTESIAN_POINT('',(32.5,0.,-42.5));
#8970=CARTESIAN_POINT('',(32.5,0.,-42.5));
#8971=CARTESIAN_POINT('',(42.5,0.,-32.5));
#8972=CARTESIAN_POINT('Origin',(32.5,0.,-32.5));
#8973=CARTESIAN_POINT('',(42.5,0.,32.5));
#8974=CARTESIAN_POINT('',(42.5,0.,32.5));
#8975=CARTESIAN_POINT('',(32.5,0.,42.5));
#8976=CARTESIAN_POINT('Origin',(32.5,0.,32.5));
#8977=CARTESIAN_POINT('',(-32.5,0.,42.5));
#8978=CARTESIAN_POINT('',(-32.5,0.,42.5));
#8979=CARTESIAN_POINT('',(-42.5,0.,32.5));
#8980=CARTESIAN_POINT('Origin',(-32.5,0.,32.5));
#8981=CARTESIAN_POINT('',(-42.5,0.,-32.5));
#8982=CARTESIAN_POINT('',(-35.,0.,-32.5));
#8983=CARTESIAN_POINT('Origin',(-32.5,0.,-32.5));
#8984=CARTESIAN_POINT('',(30.,0.,32.5));
#8985=CARTESIAN_POINT('Origin',(32.5,0.,32.5));
#8986=CARTESIAN_POINT('',(30.,0.,-32.5));
#8987=CARTESIAN_POINT('Origin',(32.5,0.,-32.5));
#8988=CARTESIAN_POINT('',(13.25,0.,2.14313189850787E-16));
#8989=CARTESIAN_POINT('Origin',(15.,0.,0.));
#8990=CARTESIAN_POINT('',(-16.75,0.,2.14313189850787E-16));
#8991=CARTESIAN_POINT('Origin',(-15.,0.,0.));
#8992=CARTESIAN_POINT('',(-35.,0.,32.5));
#8993=CARTESIAN_POINT('Origin',(-32.5,0.,32.5));
#8994=CARTESIAN_POINT('Origin',(-32.5,0.,32.5));
#8995=CARTESIAN_POINT('',(-35.,6.,32.5));
#8996=CARTESIAN_POINT('',(-35.,0.,32.5));
#8997=CARTESIAN_POINT('Origin',(-32.5,6.,32.5));
#8998=CARTESIAN_POINT('Origin',(0.,6.,0.));
#8999=CARTESIAN_POINT('',(40.4999999999501,6.00000000004757,-32.4999999910564));
#9000=CARTESIAN_POINT('',(32.4999999901967,6.0000000000829,-40.4999999999151));
#9001=CARTESIAN_POINT('Origin',(32.5,6.,-32.5));
#9002=CARTESIAN_POINT('',(-32.4999999897,6.000000000096,-40.4999999999));
#9003=CARTESIAN_POINT('',(32.49999998871,6.000000000167,-40.49999999983));
#9004=CARTESIAN_POINT('',(-40.4999999999151,6.0000000000829,-32.4999999901967));
#9005=CARTESIAN_POINT('Origin',(-32.5,6.,-32.5));
#9006=CARTESIAN_POINT('',(-40.4999999999,6.000000000096,32.4999999897));
#9007=CARTESIAN_POINT('',(-40.49999999983,6.000000000167,-32.49999998871));
#9008=CARTESIAN_POINT('',(-32.4999999901967,6.0000000000829,40.4999999999151));
#9009=CARTESIAN_POINT('Origin',(-32.5,6.,32.5));
#9010=CARTESIAN_POINT('',(32.4999999897,6.000000000096,40.4999999999));
#9011=CARTESIAN_POINT('',(-32.49999998871,6.000000000167,40.49999999983));
#9012=CARTESIAN_POINT('',(40.4999999999151,6.0000000000829,32.4999999901967));
#9013=CARTESIAN_POINT('Origin',(32.5,6.,32.5));
#9014=CARTESIAN_POINT('',(40.49999999983,6.000000000167,32.49999998871));
#9015=CARTESIAN_POINT('',(-35.,6.,-32.5));
#9016=CARTESIAN_POINT('Origin',(-32.5,6.,-32.5));
#9017=CARTESIAN_POINT('',(30.,6.,32.5));
#9018=CARTESIAN_POINT('Origin',(32.5,6.,32.5));
#9019=CARTESIAN_POINT('',(30.,6.,-32.5));
#9020=CARTESIAN_POINT('Origin',(32.5,6.,-32.5));
#9021=CARTESIAN_POINT('',(13.25,6.,2.14313189850787E-16));
#9022=CARTESIAN_POINT('Origin',(15.,6.,0.));
#9023=CARTESIAN_POINT('',(-16.75,6.,2.14313189850787E-16));
#9024=CARTESIAN_POINT('Origin',(-15.,6.,0.));
#9025=CARTESIAN_POINT('Origin',(-32.5,0.,-32.5));
#9026=CARTESIAN_POINT('',(-35.,0.,-32.5));
#9027=CARTESIAN_POINT('Origin',(32.5,0.,32.5));
#9028=CARTESIAN_POINT('',(30.,0.,32.5));
#9029=CARTESIAN_POINT('Origin',(32.5,0.,-32.5));
#9030=CARTESIAN_POINT('',(30.,0.,-32.5));
#9031=CARTESIAN_POINT('Origin',(15.,0.,0.));
#9032=CARTESIAN_POINT('',(13.25,0.,2.14313189850787E-16));
#9033=CARTESIAN_POINT('Origin',(-15.,0.,0.));
#9034=CARTESIAN_POINT('',(-16.75,0.,2.14313189850787E-16));
#9035=CARTESIAN_POINT('Origin',(32.5,5.000000000251,-32.5));
#9036=CARTESIAN_POINT('',(42.4999999999408,4.00000000004547,-32.4999999909456));
#9037=CARTESIAN_POINT('',(40.4999999999,6.000000000096,-32.4999999897));
#9038=CARTESIAN_POINT('',(32.4999999900768,4.00000000007925,-42.4999999998988));
#9039=CARTESIAN_POINT('Origin',(32.5,4.,-32.5));
#9040=CARTESIAN_POINT('',(32.49999998871,6.000000000167,-40.49999999983));
#9041=CARTESIAN_POINT('Origin',(1.24344978758E-14,5.,-41.5));
#9042=CARTESIAN_POINT('',(-32.49999999034,4.00000000009,-42.49999999991));
#9043=CARTESIAN_POINT('',(32.49999998941,4.000000000157,-42.49999999984));
#9044=CARTESIAN_POINT('',(-32.4999999897,6.000000000096,-40.4999999999));
#9045=CARTESIAN_POINT('Origin',(-32.5,5.000000000251,-32.5));
#9046=CARTESIAN_POINT('',(-42.4999999998987,4.0000000000792,-32.4999999900768));
#9047=CARTESIAN_POINT('Origin',(-32.5,4.,-32.5));
#9048=CARTESIAN_POINT('',(-40.49999999983,6.000000000167,-32.49999998871));
#9049=CARTESIAN_POINT('Origin',(-41.5,5.,-1.24344978758E-14));
#9050=CARTESIAN_POINT('',(-42.49999999991,4.00000000009,32.49999999034));
#9051=CARTESIAN_POINT('',(-42.49999999984,4.000000000157,-32.49999998941));
#9052=CARTESIAN_POINT('',(-40.4999999999,6.000000000096,32.4999999897));
#9053=CARTESIAN_POINT('Origin',(-32.5,5.000000000251,32.5));
#9054=CARTESIAN_POINT('',(-32.4999999900768,4.00000000007925,42.4999999998988));
#9055=CARTESIAN_POINT('Origin',(-32.5,4.,32.5));
#9056=CARTESIAN_POINT('',(-32.49999998871,6.000000000167,40.49999999983));
#9057=CARTESIAN_POINT('Origin',(-1.24344978758E-14,5.,41.5));
#9058=CARTESIAN_POINT('',(32.49999999034,4.00000000009,42.49999999991));
#9059=CARTESIAN_POINT('',(-32.49999998941,4.000000000157,42.49999999984));
#9060=CARTESIAN_POINT('',(32.4999999897,6.000000000096,40.4999999999));
#9061=CARTESIAN_POINT('Origin',(32.5,5.000000000251,32.5));
#9062=CARTESIAN_POINT('',(42.4999999998987,4.0000000000792,32.4999999900768));
#9063=CARTESIAN_POINT('Origin',(32.5,4.,32.5));
#9064=CARTESIAN_POINT('',(40.49999999983,6.000000000167,32.49999998871));
#9065=CARTESIAN_POINT('Origin',(41.5,5.,1.24344978758E-14));
#9066=CARTESIAN_POINT('',(42.49999999984,4.000000000157,32.49999998941));
#9067=CARTESIAN_POINT('Origin',(42.5,0.,32.5));
#9068=CARTESIAN_POINT('',(42.5,0.,32.5));
#9069=CARTESIAN_POINT('',(42.5,0.,-32.5));
#9070=CARTESIAN_POINT('Origin',(32.5,0.,-32.5));
#9071=CARTESIAN_POINT('',(32.5,0.,-42.5));
#9072=CARTESIAN_POINT('Origin',(32.5,0.,-42.5));
#9073=CARTESIAN_POINT('',(-32.5,0.,-42.5));
#9074=CARTESIAN_POINT('Origin',(-32.5,0.,-32.5));
#9075=CARTESIAN_POINT('',(-42.5,0.,-32.5));
#9076=CARTESIAN_POINT('Origin',(-42.5,0.,-32.5));
#9077=CARTESIAN_POINT('',(-42.5,0.,32.5));
#9078=CARTESIAN_POINT('Origin',(-32.5,0.,32.5));
#9079=CARTESIAN_POINT('',(-32.5,0.,42.5));
#9080=CARTESIAN_POINT('Origin',(-32.5,0.,42.5));
#9081=CARTESIAN_POINT('',(32.5,0.,42.5));
#9082=CARTESIAN_POINT('Origin',(32.5,0.,32.5));
#9083=CARTESIAN_POINT('Origin',(-15.,6.,0.));
#9084=CARTESIAN_POINT('',(-13.,6.,-2.44929359829471E-16));
#9085=CARTESIAN_POINT('Origin',(-15.,6.,0.));
#9086=CARTESIAN_POINT('',(-13.,0.,-2.44929359829471E-16));
#9087=CARTESIAN_POINT('',(-13.,6.,-2.44929359829471E-16));
#9088=CARTESIAN_POINT('Origin',(-15.,0.,0.));
#9089=CARTESIAN_POINT('Origin',(-15.,0.,0.));
#9090=CARTESIAN_POINT('',(-16.75,0.,0.));
#9091=CARTESIAN_POINT('Origin',(-15.,0.,0.));
#9092=CARTESIAN_POINT('Origin',(15.,6.,0.));
#9093=CARTESIAN_POINT('',(17.,6.,-2.44929359829471E-16));
#9094=CARTESIAN_POINT('Origin',(15.,6.,0.));
#9095=CARTESIAN_POINT('',(17.,0.,-2.44929359829471E-16));
#9096=CARTESIAN_POINT('',(17.,6.,-2.44929359829471E-16));
#9097=CARTESIAN_POINT('Origin',(15.,0.,0.));
#9098=CARTESIAN_POINT('Origin',(15.,0.,0.));
#9099=CARTESIAN_POINT('',(13.25,0.,0.));
#9100=CARTESIAN_POINT('Origin',(15.,0.,0.));
#17071=UNCERTAINTY_MEASURE_WITH_UNIT(LENGTH_MEASURE(0.01),#17114,
'DISTANCE_ACCURACY_VALUE',
'Maximum model space distance between geometric entities at asserted c
onnectivities');
#17090=UNCERTAINTY_MEASURE_WITH_UNIT(LENGTH_MEASURE(0.01),#17114,
'DISTANCE_ACCURACY_VALUE',
'Maximum model space distance between geometric entities at asserted c
onnectivities');
#17094=(
GEOMETRIC_REPRESENTATION_CONTEXT(3)
GLOBAL_UNCERTAINTY_ASSIGNED_CONTEXT((#17071))
GLOBAL_UNIT_ASSIGNED_CONTEXT((#17114,#17116,#17117))
REPRESENTATION_CONTEXT('','3D')
);
#17113=(
GEOMETRIC_REPRESENTATION_CONTEXT(3)
GLOBAL_UNCERTAINTY_ASSIGNED_CONTEXT((#17090))
GLOBAL_UNIT_ASSIGNED_CONTEXT((#17114,#17116,#17117))
REPRESENTATION_CONTEXT('','3D')
);
#17114=(
LENGTH_UNIT()
NAMED_UNIT(*)
SI_UNIT(.MILLI.,.METRE.)
);
#17116=(
NAMED_UNIT(*)
PLANE_ANGLE_UNIT()
SI_UNIT($,.RADIAN.)
);
#17117=(
NAMED_UNIT(*)
SI_UNIT($,.STERADIAN.)
SOLID_ANGLE_UNIT()
);
#17121=SHAPE_DEFINITION_REPRESENTATION(#17143,#17187);
#17143=PRODUCT_DEFINITION_SHAPE('',$,#17210);
#17187=SHAPE_REPRESENTATION('',(#6242,#239,#240),#17094);
#17206=PRODUCT_DEFINITION_CONTEXT('part definition',#17274,'design');
#17210=PRODUCT_DEFINITION('BASEPLATE','BASEPLATE',#17232,#17206);
#17232=PRODUCT_DEFINITION_FORMATION('',$,#17279);
#17274=APPLICATION_CONTEXT(
'Core Data for Automotive Mechanical Design Process');
#17275=PRODUCT_CONTEXT('part definition',#17274,'mechanical');
#17279=PRODUCT('BASEPLATE','BASEPLATE','NOT SPECIFIED',(#17275));
#17298=PRESENTATION_STYLE_ASSIGNMENT((#17299));
#17299=SURFACE_STYLE_USAGE(.BOTH.,#17300);
#17300=SURFACE_SIDE_STYLE('',(#17301));
#17301=SURFACE_STYLE_FILL_AREA(#17302);
#17302=FILL_AREA_STYLE('Steel - Satin',(#17303));
#17303=FILL_AREA_STYLE_COLOUR('Steel - Satin',#17304);
#17304=COLOUR_RGB('Steel - Satin', 0.09019608, 0.27058824, 0.51372549);
ENDSEC;
END-ISO-10303-21;
